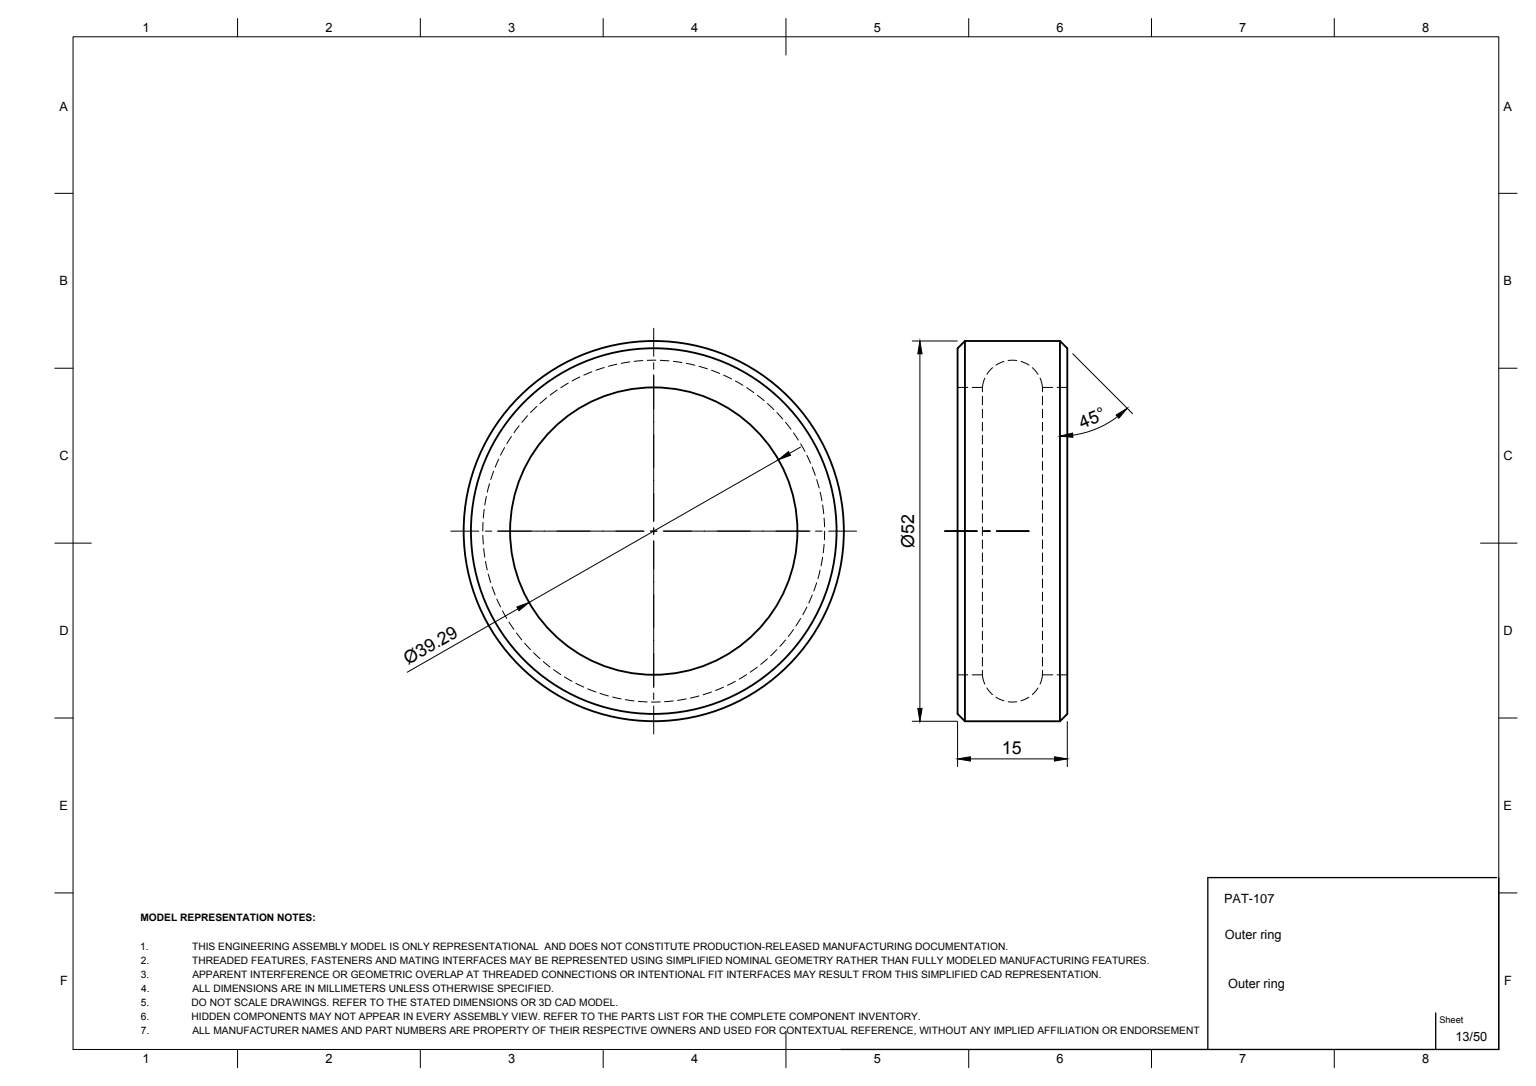
ISO-10303-21;
HEADER;
/* Generated by software containing ST-Developer
 * from STEP Tools, Inc. (www.steptools.com) 
 */

FILE_DESCRIPTION(
/* description */ ('Turntable on roller ring'),
/* implementation_level */ '2;1');

FILE_NAME(
/* name */ 'Outer ring.step',
/* time_stamp */ '2026-10-28T03:23:59-07:00',
/* author */ (''),
/* organization */ (''),
/* preprocessor_version */ 'ST-DEVELOPER v20.2',
/* originating_system */ 'Autodesk Translation Framework v15.17.0.0',
/* authorisation */ '');

FILE_SCHEMA (('AUTOMOTIVE_DESIGN { 1 0 10303 214 3 1 1 }'));
ENDSEC;

DATA;
#10=MECHANICAL_DESIGN_GEOMETRIC_PRESENTATION_REPRESENTATION('',(#622),#16281);
#473=TOROIDAL_SURFACE('',#9252,1.925,0.412776);
#481=CONICAL_SURFACE('',#9263,2.55,0.785398163397449);
#482=CONICAL_SURFACE('',#9267,2.55,0.785398163397449);
#512=SHAPE_REPRESENTATION_RELATIONSHIP('SRR','None',#16527,#567);
#567=ADVANCED_BREP_SHAPE_REPRESENTATION('',(#693),#16221);
#622=STYLED_ITEM('',(#16932),#693);
#693=MANIFOLD_SOLID_BREP('Body1',#8364);
#826=FACE_BOUND('',#1917,.T.);
#827=FACE_BOUND('',#1922,.T.);
#1023=PLANE('',#9260);
#1024=PLANE('',#9269);
#1340=FACE_OUTER_BOUND('',#1914,.T.);
#1341=FACE_OUTER_BOUND('',#1915,.T.);
#1342=FACE_OUTER_BOUND('',#1916,.T.);
#1343=FACE_OUTER_BOUND('',#1918,.T.);
#1344=FACE_OUTER_BOUND('',#1919,.T.);
#1345=FACE_OUTER_BOUND('',#1920,.T.);
#1346=FACE_OUTER_BOUND('',#1921,.T.);
#1347=FACE_OUTER_BOUND('',#1923,.T.);
#1914=EDGE_LOOP('',(#6051,#6052,#6053,#6054,#6055,#6056));
#1915=EDGE_LOOP('',(#6057,#6058,#6059,#6060,#6061));
#1916=EDGE_LOOP('',(#6062));
#1917=EDGE_LOOP('',(#6063));
#1918=EDGE_LOOP('',(#6064,#6065,#6066,#6067));
#1919=EDGE_LOOP('',(#6068,#6069,#6070,#6071));
#1920=EDGE_LOOP('',(#6072,#6073,#6074,#6075));
#1921=EDGE_LOOP('',(#6076));
#1922=EDGE_LOOP('',(#6077));
#1923=EDGE_LOOP('',(#6078,#6079,#6080,#6081,#6082));
#2583=LINE('',#13446,#3066);
#2584=LINE('',#13455,#3067);
#2585=LINE('',#13459,#3068);
#2586=LINE('',#13463,#3069);
#2587=LINE('',#13466,#3070);
#3066=VECTOR('',#10730,1.96469);
#3067=VECTOR('',#10741,2.55);
#3068=VECTOR('',#10746,2.6);
#3069=VECTOR('',#10751,2.55);
#3070=VECTOR('',#10756,1.96469);
#3572=CIRCLE('',#9253,1.96469);
#3573=CIRCLE('',#9254,1.96469);
#3574=CIRCLE('',#9255,0.412776);
#3575=CIRCLE('',#9256,1.96469);
#3576=CIRCLE('',#9257,1.96469);
#3577=CIRCLE('',#9259,1.96469);
#3578=CIRCLE('',#9261,2.5);
#3579=CIRCLE('',#9262,1.96469);
#3580=CIRCLE('',#9264,2.6);
#3581=CIRCLE('',#9266,2.6);
#3582=CIRCLE('',#9268,2.5);
#4077=VERTEX_POINT('',#13434);
#4078=VERTEX_POINT('',#13435);
#4079=VERTEX_POINT('',#13438);
#4080=VERTEX_POINT('',#13440);
#4081=VERTEX_POINT('',#13444);
#4082=VERTEX_POINT('',#13448);
#4083=VERTEX_POINT('',#13450);
#4084=VERTEX_POINT('',#13453);
#4085=VERTEX_POINT('',#13457);
#4086=VERTEX_POINT('',#13461);
#4836=EDGE_CURVE('',#4077,#4078,#3572,.T.);
#4837=EDGE_CURVE('',#4078,#4077,#3573,.T.);
#4838=EDGE_CURVE('',#4078,#4079,#3574,.T.);
#4839=EDGE_CURVE('',#4080,#4079,#3575,.T.);
#4840=EDGE_CURVE('',#4079,#4080,#3576,.T.);
#4841=EDGE_CURVE('',#4081,#4081,#3577,.T.);
#4842=EDGE_CURVE('',#4081,#4080,#2583,.T.);
#4843=EDGE_CURVE('',#4082,#4082,#3578,.T.);
#4844=EDGE_CURVE('',#4083,#4083,#3579,.T.);
#4845=EDGE_CURVE('',#4084,#4084,#3580,.T.);
#4846=EDGE_CURVE('',#4084,#4082,#2584,.T.);
#4847=EDGE_CURVE('',#4085,#4085,#3581,.T.);
#4848=EDGE_CURVE('',#4085,#4084,#2585,.T.);
#4849=EDGE_CURVE('',#4086,#4086,#3582,.T.);
#4850=EDGE_CURVE('',#4086,#4085,#2586,.T.);
#4851=EDGE_CURVE('',#4077,#4083,#2587,.T.);
#6051=ORIENTED_EDGE('',*,*,#4836,.F.);
#6052=ORIENTED_EDGE('',*,*,#4837,.F.);
#6053=ORIENTED_EDGE('',*,*,#4838,.T.);
#6054=ORIENTED_EDGE('',*,*,#4839,.F.);
#6055=ORIENTED_EDGE('',*,*,#4840,.F.);
#6056=ORIENTED_EDGE('',*,*,#4838,.F.);
#6057=ORIENTED_EDGE('',*,*,#4841,.T.);
#6058=ORIENTED_EDGE('',*,*,#4842,.T.);
#6059=ORIENTED_EDGE('',*,*,#4839,.T.);
#6060=ORIENTED_EDGE('',*,*,#4840,.T.);
#6061=ORIENTED_EDGE('',*,*,#4842,.F.);
#6062=ORIENTED_EDGE('',*,*,#4843,.F.);
#6063=ORIENTED_EDGE('',*,*,#4844,.T.);
#6064=ORIENTED_EDGE('',*,*,#4845,.F.);
#6065=ORIENTED_EDGE('',*,*,#4846,.T.);
#6066=ORIENTED_EDGE('',*,*,#4843,.T.);
#6067=ORIENTED_EDGE('',*,*,#4846,.F.);
#6068=ORIENTED_EDGE('',*,*,#4847,.F.);
#6069=ORIENTED_EDGE('',*,*,#4848,.T.);
#6070=ORIENTED_EDGE('',*,*,#4845,.T.);
#6071=ORIENTED_EDGE('',*,*,#4848,.F.);
#6072=ORIENTED_EDGE('',*,*,#4849,.F.);
#6073=ORIENTED_EDGE('',*,*,#4850,.T.);
#6074=ORIENTED_EDGE('',*,*,#4847,.T.);
#6075=ORIENTED_EDGE('',*,*,#4850,.F.);
#6076=ORIENTED_EDGE('',*,*,#4849,.T.);
#6077=ORIENTED_EDGE('',*,*,#4841,.F.);
#6078=ORIENTED_EDGE('',*,*,#4836,.T.);
#6079=ORIENTED_EDGE('',*,*,#4837,.T.);
#6080=ORIENTED_EDGE('',*,*,#4851,.T.);
#6081=ORIENTED_EDGE('',*,*,#4844,.F.);
#6082=ORIENTED_EDGE('',*,*,#4851,.F.);
#7720=CYLINDRICAL_SURFACE('',#9258,1.96469);
#7721=CYLINDRICAL_SURFACE('',#9265,2.6);
#7722=CYLINDRICAL_SURFACE('',#9270,1.96469);
#7943=ADVANCED_FACE('',(#1340),#473,.F.);
#7944=ADVANCED_FACE('',(#1341),#7720,.F.);
#7945=ADVANCED_FACE('',(#1342,#826),#1023,.T.);
#7946=ADVANCED_FACE('',(#1343),#481,.T.);
#7947=ADVANCED_FACE('',(#1344),#7721,.T.);
#7948=ADVANCED_FACE('',(#1345),#482,.T.);
#7949=ADVANCED_FACE('',(#1346,#827),#1024,.T.);
#7950=ADVANCED_FACE('',(#1347),#7722,.F.);
#8364=CLOSED_SHELL('',(#7943,#7944,#7945,#7946,#7947,#7948,#7949,#7950));
#9251=AXIS2_PLACEMENT_3D('',#13432,#10712,#10713);
#9252=AXIS2_PLACEMENT_3D('',#13433,#10714,#10715);
#9253=AXIS2_PLACEMENT_3D('',#13436,#10716,#10717);
#9254=AXIS2_PLACEMENT_3D('',#13437,#10718,#10719);
#9255=AXIS2_PLACEMENT_3D('',#13439,#10720,#10721);
#9256=AXIS2_PLACEMENT_3D('',#13441,#10722,#10723);
#9257=AXIS2_PLACEMENT_3D('',#13442,#10724,#10725);
#9258=AXIS2_PLACEMENT_3D('',#13443,#10726,#10727);
#9259=AXIS2_PLACEMENT_3D('',#13445,#10728,#10729);
#9260=AXIS2_PLACEMENT_3D('',#13447,#10731,#10732);
#9261=AXIS2_PLACEMENT_3D('',#13449,#10733,#10734);
#9262=AXIS2_PLACEMENT_3D('',#13451,#10735,#10736);
#9263=AXIS2_PLACEMENT_3D('',#13452,#10737,#10738);
#9264=AXIS2_PLACEMENT_3D('',#13454,#10739,#10740);
#9265=AXIS2_PLACEMENT_3D('',#13456,#10742,#10743);
#9266=AXIS2_PLACEMENT_3D('',#13458,#10744,#10745);
#9267=AXIS2_PLACEMENT_3D('',#13460,#10747,#10748);
#9268=AXIS2_PLACEMENT_3D('',#13462,#10749,#10750);
#9269=AXIS2_PLACEMENT_3D('',#13464,#10752,#10753);
#9270=AXIS2_PLACEMENT_3D('',#13465,#10754,#10755);
#10712=DIRECTION('axis',(0.,0.,1.));
#10713=DIRECTION('refdir',(1.,0.,0.));
#10714=DIRECTION('center_axis',(0.,-1.,0.));
#10715=DIRECTION('ref_axis',(0.,0.,-1.));
#10716=DIRECTION('center_axis',(0.,-1.,0.));
#10717=DIRECTION('ref_axis',(1.,0.,0.));
#10718=DIRECTION('center_axis',(0.,-1.,0.));
#10719=DIRECTION('ref_axis',(1.,0.,0.));
#10720=DIRECTION('center_axis',(1.,0.,1.22464679914735E-16));
#10721=DIRECTION('ref_axis',(-1.22464679914735E-16,0.,1.));
#10722=DIRECTION('center_axis',(0.,1.,0.));
#10723=DIRECTION('ref_axis',(1.,0.,0.));
#10724=DIRECTION('center_axis',(0.,1.,0.));
#10725=DIRECTION('ref_axis',(1.,0.,0.));
#10726=DIRECTION('center_axis',(0.,-1.,0.));
#10727=DIRECTION('ref_axis',(1.,0.,0.));
#10728=DIRECTION('center_axis',(0.,-1.,0.));
#10729=DIRECTION('ref_axis',(1.,0.,0.));
#10730=DIRECTION('',(0.,1.,0.));
#10731=DIRECTION('center_axis',(0.,1.,0.));
#10732=DIRECTION('ref_axis',(0.,0.,1.));
#10733=DIRECTION('center_axis',(0.,-1.,0.));
#10734=DIRECTION('ref_axis',(1.,0.,0.));
#10735=DIRECTION('center_axis',(0.,-1.,0.));
#10736=DIRECTION('ref_axis',(1.,0.,0.));
#10737=DIRECTION('center_axis',(0.,-1.,0.));
#10738=DIRECTION('ref_axis',(1.,0.,0.));
#10739=DIRECTION('center_axis',(0.,-1.,0.));
#10740=DIRECTION('ref_axis',(1.,0.,0.));
#10741=DIRECTION('',(0.707106781186548,0.707106781186547,8.65956056235494E-17));
#10742=DIRECTION('center_axis',(0.,-1.,0.));
#10743=DIRECTION('ref_axis',(1.,0.,0.));
#10744=DIRECTION('center_axis',(0.,-1.,0.));
#10745=DIRECTION('ref_axis',(1.,0.,0.));
#10746=DIRECTION('',(0.,1.,0.));
#10747=DIRECTION('center_axis',(0.,1.,0.));
#10748=DIRECTION('ref_axis',(1.,0.,0.));
#10749=DIRECTION('center_axis',(0.,-1.,0.));
#10750=DIRECTION('ref_axis',(1.,0.,0.));
#10751=DIRECTION('',(-0.707106781186548,0.707106781186547,-8.65956056235494E-17));
#10752=DIRECTION('center_axis',(0.,-1.,0.));
#10753=DIRECTION('ref_axis',(0.,0.,-1.));
#10754=DIRECTION('center_axis',(0.,-1.,0.));
#10755=DIRECTION('ref_axis',(1.,0.,0.));
#10756=DIRECTION('',(0.,1.,0.));
#13432=CARTESIAN_POINT('',(0.,0.,0.));
#13433=CARTESIAN_POINT('Origin',(0.,0.,0.));
#13434=CARTESIAN_POINT('',(-1.96469,0.410863395882378,-2.40605131981681E-16));
#13435=CARTESIAN_POINT('',(-2.40605131981681E-16,0.410863395882378,1.96469));
#13436=CARTESIAN_POINT('Origin',(0.,0.410863395882378,0.));
#13437=CARTESIAN_POINT('Origin',(0.,0.410863395882378,0.));
#13438=CARTESIAN_POINT('',(-2.40605131981681E-16,-0.410863395882378,1.96469));
#13439=CARTESIAN_POINT('Origin',(-2.35744508835865E-16,0.,1.925));
#13440=CARTESIAN_POINT('',(-1.96469,-0.410863395882378,2.40605131981681E-16));
#13441=CARTESIAN_POINT('Origin',(0.,-0.410863395882378,0.));
#13442=CARTESIAN_POINT('Origin',(0.,-0.410863395882378,0.));
#13443=CARTESIAN_POINT('Origin',(0.,0.,0.));
#13444=CARTESIAN_POINT('',(-1.96469,-0.75,-2.40605131981681E-16));
#13445=CARTESIAN_POINT('Origin',(0.,-0.75,0.));
#13446=CARTESIAN_POINT('',(-1.96469,0.,-2.40605131981681E-16));
#13447=CARTESIAN_POINT('Origin',(2.5,0.75,0.));
#13448=CARTESIAN_POINT('',(-2.5,0.75,-3.06161699786838E-16));
#13449=CARTESIAN_POINT('Origin',(0.,0.75,0.));
#13450=CARTESIAN_POINT('',(-1.96469,0.75,-2.40605131981681E-16));
#13451=CARTESIAN_POINT('Origin',(0.,0.75,0.));
#13452=CARTESIAN_POINT('Origin',(0.,0.7,0.));
#13453=CARTESIAN_POINT('',(-2.6,0.65,-3.18408167778312E-16));
#13454=CARTESIAN_POINT('Origin',(0.,0.65,0.));
#13455=CARTESIAN_POINT('',(-2.55,0.7,-3.12284933782575E-16));
#13456=CARTESIAN_POINT('Origin',(0.,0.,0.));
#13457=CARTESIAN_POINT('',(-2.6,-0.65,-3.18408167778312E-16));
#13458=CARTESIAN_POINT('Origin',(0.,-0.65,0.));
#13459=CARTESIAN_POINT('',(-2.6,0.,-3.18408167778312E-16));
#13460=CARTESIAN_POINT('Origin',(0.,-0.7,0.));
#13461=CARTESIAN_POINT('',(-2.5,-0.75,-3.06161699786838E-16));
#13462=CARTESIAN_POINT('Origin',(0.,-0.75,0.));
#13463=CARTESIAN_POINT('',(-2.55,-0.7,-3.12284933782575E-16));
#13464=CARTESIAN_POINT('Origin',(1.96469,-0.75,0.));
#13465=CARTESIAN_POINT('Origin',(0.,0.,0.));
#13466=CARTESIAN_POINT('',(-1.96469,0.,-2.40605131981681E-16));
#16152=UNCERTAINTY_MEASURE_WITH_UNIT(LENGTH_MEASURE(0.001),#16282,
'DISTANCE_ACCURACY_VALUE',
'Maximum model space distance between geometric entities at asserted c
onnectivities');
#16212=UNCERTAINTY_MEASURE_WITH_UNIT(LENGTH_MEASURE(0.001),#16282,
'DISTANCE_ACCURACY_VALUE',
'Maximum model space distance between geometric entities at asserted c
onnectivities');
#16221=(
GEOMETRIC_REPRESENTATION_CONTEXT(3)
GLOBAL_UNCERTAINTY_ASSIGNED_CONTEXT((#16152))
GLOBAL_UNIT_ASSIGNED_CONTEXT((#16282,#16284,#16285))
REPRESENTATION_CONTEXT('','3D')
);
#16281=(
GEOMETRIC_REPRESENTATION_CONTEXT(3)
GLOBAL_UNCERTAINTY_ASSIGNED_CONTEXT((#16212))
GLOBAL_UNIT_ASSIGNED_CONTEXT((#16282,#16284,#16285))
REPRESENTATION_CONTEXT('','3D')
);
#16282=(
LENGTH_UNIT()
NAMED_UNIT(*)
SI_UNIT(.CENTI.,.METRE.)
);
#16284=(
NAMED_UNIT(*)
PLANE_ANGLE_UNIT()
SI_UNIT($,.RADIAN.)
);
#16285=(
NAMED_UNIT(*)
SI_UNIT($,.STERADIAN.)
SOLID_ANGLE_UNIT()
);
#16294=SHAPE_DEFINITION_REPRESENTATION(#16362,#16527);
#16362=PRODUCT_DEFINITION_SHAPE('',$,#16596);
#16527=SHAPE_REPRESENTATION('',(#9251),#16221);
#16587=PRODUCT_DEFINITION_CONTEXT('part definition',#16793,'design');
#16596=PRODUCT_DEFINITION('Outer ring','Outer ring',#16664,#16587);
#16664=PRODUCT_DEFINITION_FORMATION('',$,#16803);
#16793=APPLICATION_CONTEXT(
'Core Data for Automotive Mechanical Design Process');
#16794=PRODUCT_CONTEXT('part definition',#16793,'mechanical');
#16803=PRODUCT('Outer ring','Outer ring','Outer ring',(#16794));
#16926=COLOUR_RGB('Grey',0.48,0.52,0.57);
#16927=FILL_AREA_STYLE_COLOUR('',#16926);
#16928=FILL_AREA_STYLE('',(#16927));
#16929=SURFACE_STYLE_FILL_AREA(#16928);
#16930=SURFACE_SIDE_STYLE('',(#16929));
#16931=SURFACE_STYLE_USAGE(.BOTH.,#16930);
#16932=PRESENTATION_STYLE_ASSIGNMENT((#16931));
ENDSEC;
END-ISO-10303-21;
